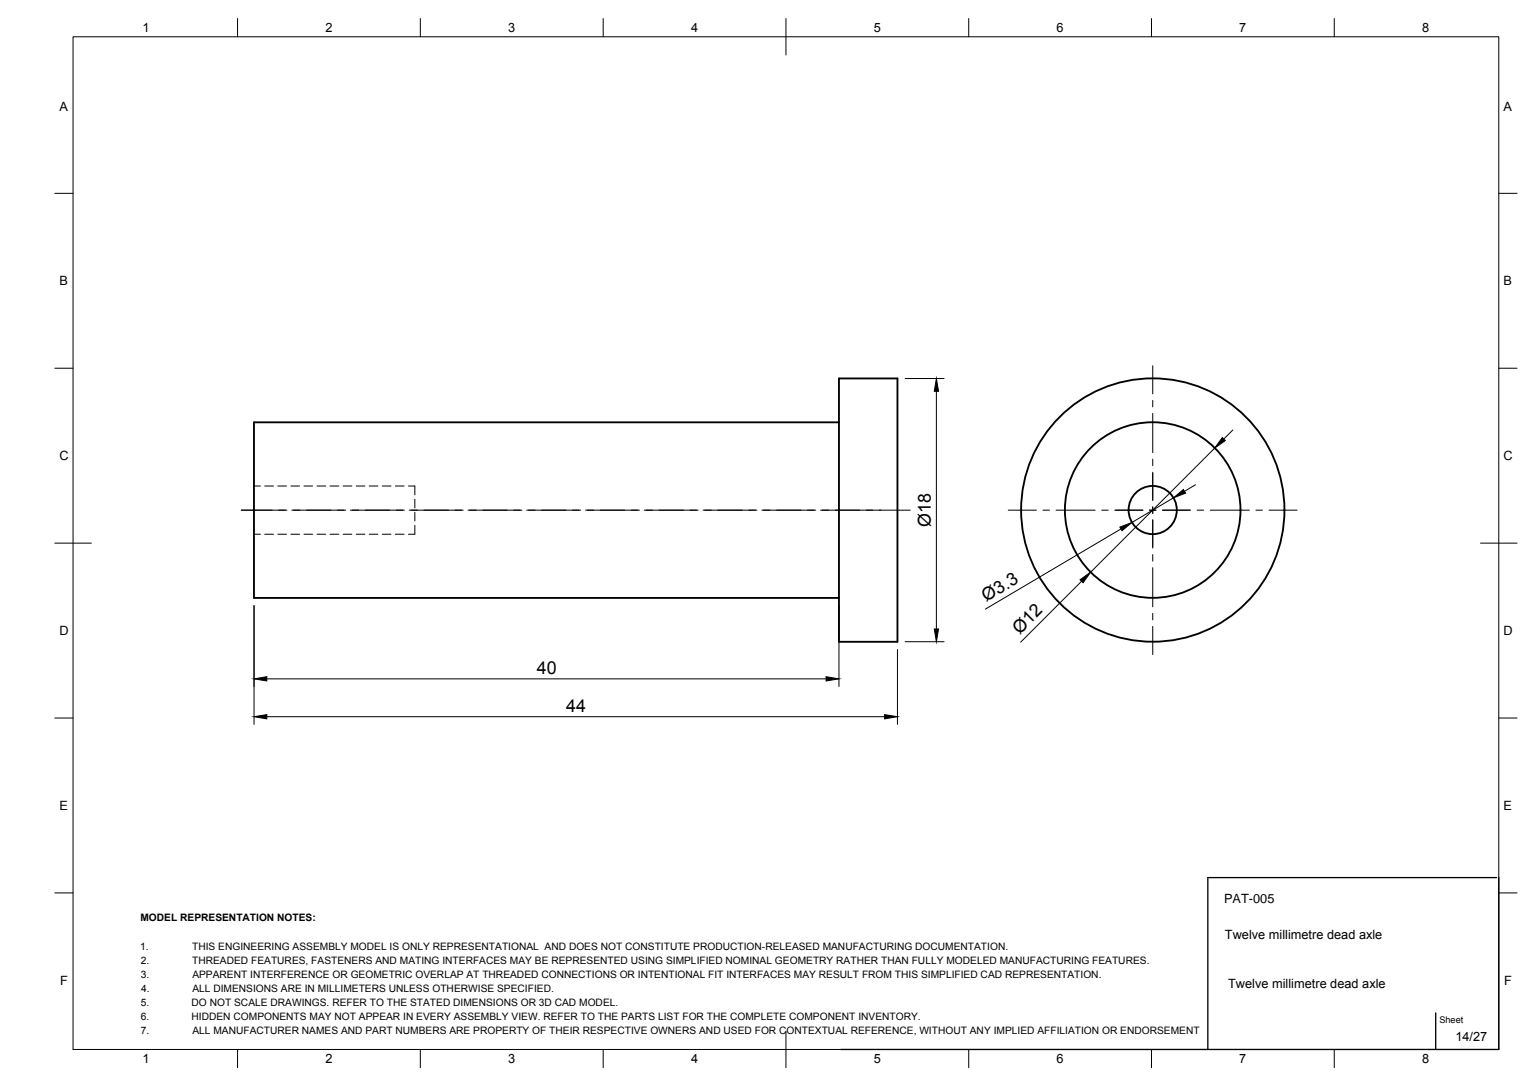
ISO-10303-21;
HEADER;
/* Generated by software containing ST-Developer
 * from STEP Tools, Inc. (www.steptools.com) 
 */

FILE_DESCRIPTION(
/* description */ ('Ball-race swivel caster'),
/* implementation_level */ '2;1');

FILE_NAME(
/* name */ 'Twelve millimetre dead axle.step',
/* time_stamp */ '2026-10-29T16:15:51-07:00',
/* author */ (''),
/* organization */ (''),
/* preprocessor_version */ 'ST-DEVELOPER v20.2',
/* originating_system */ 'Autodesk Translation Framework v15.17.0.0',
/* authorisation */ '');

FILE_SCHEMA (('AUTOMOTIVE_DESIGN { 1 0 10303 214 3 1 1 }'));
ENDSEC;

DATA;
#10=MECHANICAL_DESIGN_GEOMETRIC_PRESENTATION_REPRESENTATION('',(#316),#7816);
#267=SHAPE_REPRESENTATION_RELATIONSHIP('SRR','None',#7914,#287);
#287=ADVANCED_BREP_SHAPE_REPRESENTATION('',(#352),#7803);
#316=STYLED_ITEM('',(#8097),#352);
#352=MANIFOLD_SOLID_BREP('Body1',#3722);
#416=FACE_BOUND('',#901,.T.);
#417=FACE_BOUND('',#906,.T.);
#483=PLANE('',#4267);
#484=PLANE('',#4268);
#485=PLANE('',#4273);
#486=PLANE('',#4276);
#642=FACE_OUTER_BOUND('',#898,.T.);
#643=FACE_OUTER_BOUND('',#899,.T.);
#644=FACE_OUTER_BOUND('',#900,.T.);
#645=FACE_OUTER_BOUND('',#902,.T.);
#646=FACE_OUTER_BOUND('',#903,.T.);
#647=FACE_OUTER_BOUND('',#904,.T.);
#648=FACE_OUTER_BOUND('',#905,.T.);
#898=EDGE_LOOP('',(#3091,#3092,#3093,#3094));
#899=EDGE_LOOP('',(#3095));
#900=EDGE_LOOP('',(#3096));
#901=EDGE_LOOP('',(#3097));
#902=EDGE_LOOP('',(#3098,#3099,#3100,#3101));
#903=EDGE_LOOP('',(#3102));
#904=EDGE_LOOP('',(#3103,#3104,#3105,#3106));
#905=EDGE_LOOP('',(#3107));
#906=EDGE_LOOP('',(#3108));
#1114=LINE('',#7063,#1269);
#1115=LINE('',#7073,#1270);
#1116=LINE('',#7079,#1271);
#1269=VECTOR('',#5200,0.165);
#1270=VECTOR('',#5213,0.9);
#1271=VECTOR('',#5222,0.6);
#1483=CIRCLE('',#4265,0.165);
#1484=CIRCLE('',#4266,0.165);
#1485=CIRCLE('',#4269,0.9);
#1486=CIRCLE('',#4270,0.6);
#1487=CIRCLE('',#4272,0.9);
#1488=CIRCLE('',#4275,0.6);
#1817=VERTEX_POINT('',#7060);
#1818=VERTEX_POINT('',#7062);
#1819=VERTEX_POINT('',#7067);
#1820=VERTEX_POINT('',#7069);
#1821=VERTEX_POINT('',#7072);
#1822=VERTEX_POINT('',#7077);
#2265=EDGE_CURVE('',#1817,#1817,#1483,.T.);
#2266=EDGE_CURVE('',#1817,#1818,#1114,.T.);
#2267=EDGE_CURVE('',#1818,#1818,#1484,.T.);
#2268=EDGE_CURVE('',#1819,#1819,#1485,.T.);
#2269=EDGE_CURVE('',#1820,#1820,#1486,.T.);
#2270=EDGE_CURVE('',#1819,#1821,#1115,.T.);
#2271=EDGE_CURVE('',#1821,#1821,#1487,.T.);
#2272=EDGE_CURVE('',#1822,#1822,#1488,.T.);
#2273=EDGE_CURVE('',#1822,#1820,#1116,.T.);
#3091=ORIENTED_EDGE('',*,*,#2265,.F.);
#3092=ORIENTED_EDGE('',*,*,#2266,.T.);
#3093=ORIENTED_EDGE('',*,*,#2267,.F.);
#3094=ORIENTED_EDGE('',*,*,#2266,.F.);
#3095=ORIENTED_EDGE('',*,*,#2265,.T.);
#3096=ORIENTED_EDGE('',*,*,#2268,.T.);
#3097=ORIENTED_EDGE('',*,*,#2269,.F.);
#3098=ORIENTED_EDGE('',*,*,#2268,.F.);
#3099=ORIENTED_EDGE('',*,*,#2270,.T.);
#3100=ORIENTED_EDGE('',*,*,#2271,.T.);
#3101=ORIENTED_EDGE('',*,*,#2270,.F.);
#3102=ORIENTED_EDGE('',*,*,#2271,.F.);
#3103=ORIENTED_EDGE('',*,*,#2272,.F.);
#3104=ORIENTED_EDGE('',*,*,#2273,.T.);
#3105=ORIENTED_EDGE('',*,*,#2269,.T.);
#3106=ORIENTED_EDGE('',*,*,#2273,.F.);
#3107=ORIENTED_EDGE('',*,*,#2272,.T.);
#3108=ORIENTED_EDGE('',*,*,#2267,.T.);
#3468=CYLINDRICAL_SURFACE('',#4264,0.165);
#3469=CYLINDRICAL_SURFACE('',#4271,0.9);
#3470=CYLINDRICAL_SURFACE('',#4274,0.6);
#3613=ADVANCED_FACE('',(#642),#3468,.F.);
#3614=ADVANCED_FACE('',(#643),#483,.T.);
#3615=ADVANCED_FACE('',(#644,#416),#484,.T.);
#3616=ADVANCED_FACE('',(#645),#3469,.T.);
#3617=ADVANCED_FACE('',(#646),#485,.F.);
#3618=ADVANCED_FACE('',(#647),#3470,.T.);
#3619=ADVANCED_FACE('',(#648,#417),#486,.T.);
#3722=CLOSED_SHELL('',(#3613,#3614,#3615,#3616,#3617,#3618,#3619));
#4263=AXIS2_PLACEMENT_3D('',#7058,#5194,#5195);
#4264=AXIS2_PLACEMENT_3D('',#7059,#5196,#5197);
#4265=AXIS2_PLACEMENT_3D('',#7061,#5198,#5199);
#4266=AXIS2_PLACEMENT_3D('',#7064,#5201,#5202);
#4267=AXIS2_PLACEMENT_3D('',#7065,#5203,#5204);
#4268=AXIS2_PLACEMENT_3D('',#7066,#5205,#5206);
#4269=AXIS2_PLACEMENT_3D('',#7068,#5207,#5208);
#4270=AXIS2_PLACEMENT_3D('',#7070,#5209,#5210);
#4271=AXIS2_PLACEMENT_3D('',#7071,#5211,#5212);
#4272=AXIS2_PLACEMENT_3D('',#7074,#5214,#5215);
#4273=AXIS2_PLACEMENT_3D('',#7075,#5216,#5217);
#4274=AXIS2_PLACEMENT_3D('',#7076,#5218,#5219);
#4275=AXIS2_PLACEMENT_3D('',#7078,#5220,#5221);
#4276=AXIS2_PLACEMENT_3D('',#7080,#5223,#5224);
#5194=DIRECTION('axis',(0.,0.,1.));
#5195=DIRECTION('refdir',(1.,0.,0.));
#5196=DIRECTION('center_axis',(0.,1.,0.));
#5197=DIRECTION('ref_axis',(1.,0.,0.));
#5198=DIRECTION('center_axis',(0.,1.,0.));
#5199=DIRECTION('ref_axis',(1.,0.,0.));
#5200=DIRECTION('',(0.,1.,0.));
#5201=DIRECTION('center_axis',(0.,-1.,0.));
#5202=DIRECTION('ref_axis',(1.,0.,0.));
#5203=DIRECTION('center_axis',(0.,1.,0.));
#5204=DIRECTION('ref_axis',(1.,0.,0.));
#5205=DIRECTION('center_axis',(0.,1.,0.));
#5206=DIRECTION('ref_axis',(1.,0.,0.));
#5207=DIRECTION('center_axis',(0.,1.,0.));
#5208=DIRECTION('ref_axis',(1.,0.,0.));
#5209=DIRECTION('center_axis',(0.,1.,0.));
#5210=DIRECTION('ref_axis',(1.,0.,0.));
#5211=DIRECTION('center_axis',(0.,1.,0.));
#5212=DIRECTION('ref_axis',(1.,0.,0.));
#5213=DIRECTION('',(0.,-1.,0.));
#5214=DIRECTION('center_axis',(0.,1.,0.));
#5215=DIRECTION('ref_axis',(1.,0.,0.));
#5216=DIRECTION('center_axis',(0.,1.,0.));
#5217=DIRECTION('ref_axis',(1.,0.,0.));
#5218=DIRECTION('center_axis',(0.,1.,0.));
#5219=DIRECTION('ref_axis',(1.,0.,0.));
#5220=DIRECTION('center_axis',(0.,1.,0.));
#5221=DIRECTION('ref_axis',(1.,0.,0.));
#5222=DIRECTION('',(0.,-1.,0.));
#5223=DIRECTION('center_axis',(0.,1.,0.));
#5224=DIRECTION('ref_axis',(1.,0.,0.));
#7058=CARTESIAN_POINT('',(0.,0.,0.));
#7059=CARTESIAN_POINT('Origin',(0.,0.9,3.5));
#7060=CARTESIAN_POINT('',(-0.165,0.9,3.5));
#7061=CARTESIAN_POINT('Origin',(0.,0.9,3.5));
#7062=CARTESIAN_POINT('',(-0.165,2.,3.5));
#7063=CARTESIAN_POINT('',(-0.165,0.9,3.5));
#7064=CARTESIAN_POINT('Origin',(0.,2.,3.5));
#7065=CARTESIAN_POINT('Origin',(0.,0.9,3.5));
#7066=CARTESIAN_POINT('Origin',(0.,-2.,3.5));
#7067=CARTESIAN_POINT('',(-0.9,-2.,3.5));
#7068=CARTESIAN_POINT('Origin',(0.,-2.,3.5));
#7069=CARTESIAN_POINT('',(-0.6,-2.,3.5));
#7070=CARTESIAN_POINT('Origin',(0.,-2.,3.5));
#7071=CARTESIAN_POINT('Origin',(0.,-2.4,3.5));
#7072=CARTESIAN_POINT('',(-0.9,-2.4,3.5));
#7073=CARTESIAN_POINT('',(-0.9,-2.4,3.5));
#7074=CARTESIAN_POINT('Origin',(0.,-2.4,3.5));
#7075=CARTESIAN_POINT('Origin',(0.,-2.4,3.5));
#7076=CARTESIAN_POINT('Origin',(0.,-2.,3.5));
#7077=CARTESIAN_POINT('',(-0.6,2.,3.5));
#7078=CARTESIAN_POINT('Origin',(0.,2.,3.5));
#7079=CARTESIAN_POINT('',(-0.6,-2.,3.5));
#7080=CARTESIAN_POINT('Origin',(0.,2.,3.5));
#7776=UNCERTAINTY_MEASURE_WITH_UNIT(LENGTH_MEASURE(0.001),#7817,
'DISTANCE_ACCURACY_VALUE',
'Maximum model space distance between geometric entities at asserted c
onnectivities');
#7789=UNCERTAINTY_MEASURE_WITH_UNIT(LENGTH_MEASURE(0.001),#7817,
'DISTANCE_ACCURACY_VALUE',
'Maximum model space distance between geometric entities at asserted c
onnectivities');
#7803=(
GEOMETRIC_REPRESENTATION_CONTEXT(3)
GLOBAL_UNCERTAINTY_ASSIGNED_CONTEXT((#7776))
GLOBAL_UNIT_ASSIGNED_CONTEXT((#7817,#7819,#7820))
REPRESENTATION_CONTEXT('','3D')
);
#7816=(
GEOMETRIC_REPRESENTATION_CONTEXT(3)
GLOBAL_UNCERTAINTY_ASSIGNED_CONTEXT((#7789))
GLOBAL_UNIT_ASSIGNED_CONTEXT((#7817,#7819,#7820))
REPRESENTATION_CONTEXT('','3D')
);
#7817=(
LENGTH_UNIT()
NAMED_UNIT(*)
SI_UNIT(.CENTI.,.METRE.)
);
#7819=(
NAMED_UNIT(*)
PLANE_ANGLE_UNIT()
SI_UNIT($,.RADIAN.)
);
#7820=(
NAMED_UNIT(*)
SI_UNIT($,.STERADIAN.)
SOLID_ANGLE_UNIT()
);
#7834=SHAPE_DEFINITION_REPRESENTATION(#7868,#7914);
#7868=PRODUCT_DEFINITION_SHAPE('',$,#7941);
#7914=SHAPE_REPRESENTATION('',(#4263),#7803);
#7927=PRODUCT_DEFINITION_CONTEXT('part definition',#8007,'design');
#7941=PRODUCT_DEFINITION('Twelve millimetre dead axle',
'Twelve millimetre dead axle',#7967,#7927);
#7967=PRODUCT_DEFINITION_FORMATION('',$,#8022);
#8007=APPLICATION_CONTEXT(
'Core Data for Automotive Mechanical Design Process');
#8008=PRODUCT_CONTEXT('part definition',#8007,'mechanical');
#8022=PRODUCT('Twelve millimetre dead axle',
'Twelve millimetre dead axle','Twelve millimetre dead axle',(#8008));
#8091=COLOUR_RGB('Grey',0.48,0.52,0.57);
#8092=FILL_AREA_STYLE_COLOUR('',#8091);
#8093=FILL_AREA_STYLE('',(#8092));
#8094=SURFACE_STYLE_FILL_AREA(#8093);
#8095=SURFACE_SIDE_STYLE('',(#8094));
#8096=SURFACE_STYLE_USAGE(.BOTH.,#8095);
#8097=PRESENTATION_STYLE_ASSIGNMENT((#8096));
ENDSEC;
END-ISO-10303-21;
